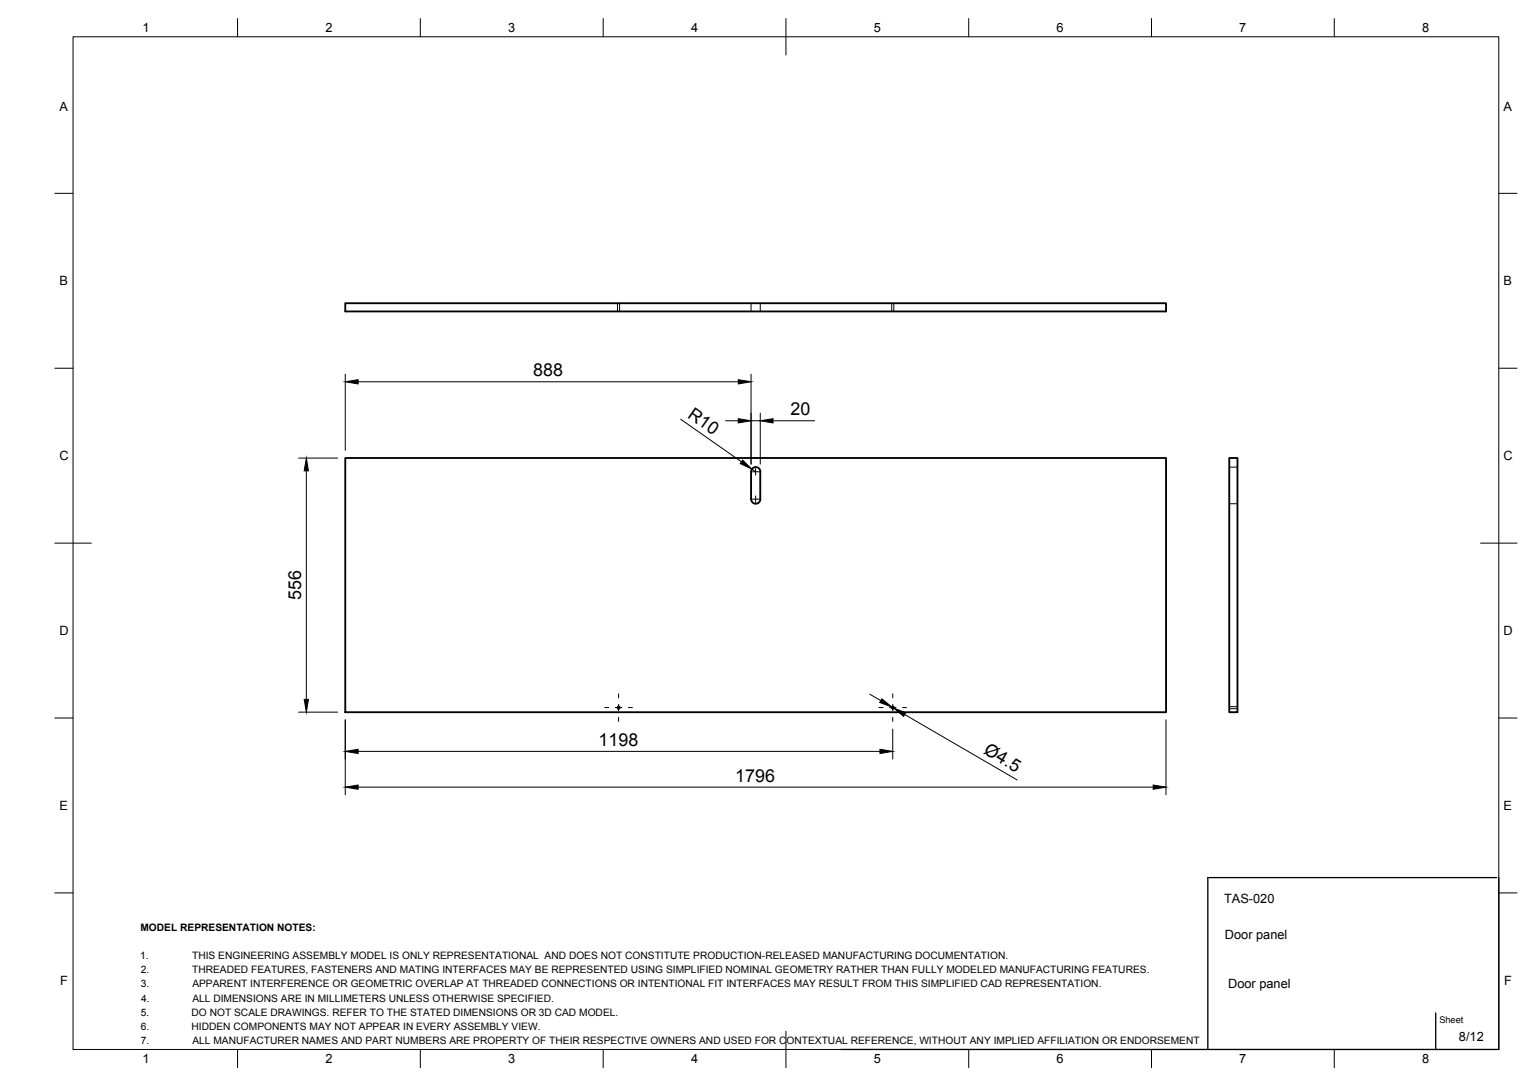
ISO-10303-21;
HEADER;
/* Generated by software containing ST-Developer
 * from STEP Tools, Inc. (www.steptools.com) 
 */

FILE_DESCRIPTION(
/* description */ (''),
/* implementation_level */ '2;1');

FILE_NAME(
/* name */ 'Door panel.step',
/* time_stamp */ '2026-11-15T17:46:57-08:00',
/* author */ (''),
/* organization */ (''),
/* preprocessor_version */ 'ST-DEVELOPER v20.2',
/* originating_system */ 'Autodesk Translation Framework v15.17.0.0',
/* authorisation */ '');

FILE_SCHEMA (('AUTOMOTIVE_DESIGN { 1 0 10303 214 3 1 1 }'));
ENDSEC;

DATA;
#10=MECHANICAL_DESIGN_GEOMETRIC_PRESENTATION_REPRESENTATION('',(#380),#12963);
#356=SHAPE_REPRESENTATION_RELATIONSHIP('SRR','None',#13040,#368);
#368=ADVANCED_BREP_SHAPE_REPRESENTATION('',(#392),#12956);
#380=STYLED_ITEM('',(#13109),#392);
#392=MANIFOLD_SOLID_BREP('Body1',#4814);
#417=FACE_BOUND('',#945,.T.);
#418=FACE_BOUND('',#946,.T.);
#419=FACE_BOUND('',#947,.T.);
#420=FACE_BOUND('',#950,.T.);
#421=FACE_BOUND('',#951,.T.);
#422=FACE_BOUND('',#952,.T.);
#519=PLANE('',#5081);
#520=PLANE('',#5085);
#521=PLANE('',#5095);
#522=PLANE('',#5096);
#523=PLANE('',#5097);
#524=PLANE('',#5098);
#525=PLANE('',#5099);
#526=PLANE('',#5100);
#664=FACE_OUTER_BOUND('',#938,.T.);
#665=FACE_OUTER_BOUND('',#939,.T.);
#666=FACE_OUTER_BOUND('',#940,.T.);
#667=FACE_OUTER_BOUND('',#941,.T.);
#668=FACE_OUTER_BOUND('',#942,.T.);
#669=FACE_OUTER_BOUND('',#943,.T.);
#670=FACE_OUTER_BOUND('',#944,.T.);
#671=FACE_OUTER_BOUND('',#948,.T.);
#672=FACE_OUTER_BOUND('',#949,.T.);
#673=FACE_OUTER_BOUND('',#953,.T.);
#674=FACE_OUTER_BOUND('',#954,.T.);
#675=FACE_OUTER_BOUND('',#955,.T.);
#938=EDGE_LOOP('',(#3544,#3545,#3546,#3547));
#939=EDGE_LOOP('',(#3548,#3549,#3550,#3551));
#940=EDGE_LOOP('',(#3552,#3553,#3554,#3555));
#941=EDGE_LOOP('',(#3556,#3557,#3558,#3559));
#942=EDGE_LOOP('',(#3560,#3561,#3562,#3563));
#943=EDGE_LOOP('',(#3564,#3565,#3566,#3567));
#944=EDGE_LOOP('',(#3568,#3569,#3570,#3571));
#945=EDGE_LOOP('',(#3572,#3573,#3574,#3575));
#946=EDGE_LOOP('',(#3576));
#947=EDGE_LOOP('',(#3577));
#948=EDGE_LOOP('',(#3578,#3579,#3580,#3581));
#949=EDGE_LOOP('',(#3582,#3583,#3584,#3585));
#950=EDGE_LOOP('',(#3586,#3587,#3588,#3589));
#951=EDGE_LOOP('',(#3590));
#952=EDGE_LOOP('',(#3591));
#953=EDGE_LOOP('',(#3592,#3593,#3594,#3595));
#954=EDGE_LOOP('',(#3596,#3597,#3598,#3599));
#955=EDGE_LOOP('',(#3600,#3601,#3602,#3603));
#1314=LINE('',#6979,#1716);
#1315=LINE('',#6981,#1717);
#1316=LINE('',#6983,#1718);
#1317=LINE('',#6984,#1719);
#1318=LINE('',#6989,#1720);
#1319=LINE('',#6993,#1721);
#1320=LINE('',#6995,#1722);
#1321=LINE('',#6996,#1723);
#1322=LINE('',#7004,#1724);
#1323=LINE('',#7010,#1725);
#1324=LINE('',#7015,#1726);
#1325=LINE('',#7017,#1727);
#1326=LINE('',#7019,#1728);
#1327=LINE('',#7020,#1729);
#1328=LINE('',#7023,#1730);
#1329=LINE('',#7025,#1731);
#1330=LINE('',#7026,#1732);
#1331=LINE('',#7029,#1733);
#1332=LINE('',#7031,#1734);
#1333=LINE('',#7032,#1735);
#1334=LINE('',#7034,#1736);
#1335=LINE('',#7035,#1737);
#1716=VECTOR('',#5785,1.);
#1717=VECTOR('',#5786,1.);
#1718=VECTOR('',#5787,1.);
#1719=VECTOR('',#5788,1.);
#1720=VECTOR('',#5793,1.);
#1721=VECTOR('',#5798,1.);
#1722=VECTOR('',#5799,1.);
#1723=VECTOR('',#5800,1.);
#1724=VECTOR('',#5811,0.225);
#1725=VECTOR('',#5818,0.225);
#1726=VECTOR('',#5823,1.);
#1727=VECTOR('',#5824,1.);
#1728=VECTOR('',#5825,1.);
#1729=VECTOR('',#5826,1.);
#1730=VECTOR('',#5829,1.);
#1731=VECTOR('',#5830,1.);
#1732=VECTOR('',#5831,1.);
#1733=VECTOR('',#5834,1.);
#1734=VECTOR('',#5835,1.);
#1735=VECTOR('',#5836,1.);
#1736=VECTOR('',#5839,1.);
#1737=VECTOR('',#5840,1.);
#1958=CIRCLE('',#5083,1.);
#1959=CIRCLE('',#5084,1.);
#1960=CIRCLE('',#5087,1.);
#1961=CIRCLE('',#5088,1.);
#1962=CIRCLE('',#5090,0.225);
#1963=CIRCLE('',#5091,0.225);
#1964=CIRCLE('',#5093,0.225);
#1965=CIRCLE('',#5094,0.225);
#2156=VERTEX_POINT('',#6977);
#2157=VERTEX_POINT('',#6978);
#2158=VERTEX_POINT('',#6980);
#2159=VERTEX_POINT('',#6982);
#2160=VERTEX_POINT('',#6986);
#2161=VERTEX_POINT('',#6988);
#2162=VERTEX_POINT('',#6992);
#2163=VERTEX_POINT('',#6994);
#2164=VERTEX_POINT('',#7001);
#2165=VERTEX_POINT('',#7003);
#2166=VERTEX_POINT('',#7007);
#2167=VERTEX_POINT('',#7009);
#2168=VERTEX_POINT('',#7013);
#2169=VERTEX_POINT('',#7014);
#2170=VERTEX_POINT('',#7016);
#2171=VERTEX_POINT('',#7018);
#2172=VERTEX_POINT('',#7022);
#2173=VERTEX_POINT('',#7024);
#2174=VERTEX_POINT('',#7028);
#2175=VERTEX_POINT('',#7030);
#2668=EDGE_CURVE('',#2156,#2157,#1314,.T.);
#2669=EDGE_CURVE('',#2156,#2158,#1315,.T.);
#2670=EDGE_CURVE('',#2159,#2158,#1316,.T.);
#2671=EDGE_CURVE('',#2157,#2159,#1317,.T.);
#2672=EDGE_CURVE('',#2160,#2156,#1958,.T.);
#2673=EDGE_CURVE('',#2160,#2161,#1318,.T.);
#2674=EDGE_CURVE('',#2158,#2161,#1959,.T.);
#2675=EDGE_CURVE('',#2162,#2160,#1319,.T.);
#2676=EDGE_CURVE('',#2162,#2163,#1320,.T.);
#2677=EDGE_CURVE('',#2161,#2163,#1321,.T.);
#2678=EDGE_CURVE('',#2157,#2162,#1960,.T.);
#2679=EDGE_CURVE('',#2163,#2159,#1961,.T.);
#2680=EDGE_CURVE('',#2164,#2164,#1962,.T.);
#2681=EDGE_CURVE('',#2164,#2165,#1322,.T.);
#2682=EDGE_CURVE('',#2165,#2165,#1963,.T.);
#2683=EDGE_CURVE('',#2166,#2166,#1964,.T.);
#2684=EDGE_CURVE('',#2166,#2167,#1323,.T.);
#2685=EDGE_CURVE('',#2167,#2167,#1965,.T.);
#2686=EDGE_CURVE('',#2168,#2169,#1324,.T.);
#2687=EDGE_CURVE('',#2169,#2170,#1325,.T.);
#2688=EDGE_CURVE('',#2171,#2170,#1326,.T.);
#2689=EDGE_CURVE('',#2168,#2171,#1327,.T.);
#2690=EDGE_CURVE('',#2172,#2168,#1328,.T.);
#2691=EDGE_CURVE('',#2173,#2171,#1329,.T.);
#2692=EDGE_CURVE('',#2172,#2173,#1330,.T.);
#2693=EDGE_CURVE('',#2174,#2172,#1331,.T.);
#2694=EDGE_CURVE('',#2175,#2173,#1332,.T.);
#2695=EDGE_CURVE('',#2174,#2175,#1333,.T.);
#2696=EDGE_CURVE('',#2169,#2174,#1334,.T.);
#2697=EDGE_CURVE('',#2170,#2175,#1335,.T.);
#3544=ORIENTED_EDGE('',*,*,#2668,.F.);
#3545=ORIENTED_EDGE('',*,*,#2669,.T.);
#3546=ORIENTED_EDGE('',*,*,#2670,.F.);
#3547=ORIENTED_EDGE('',*,*,#2671,.F.);
#3548=ORIENTED_EDGE('',*,*,#2672,.F.);
#3549=ORIENTED_EDGE('',*,*,#2673,.T.);
#3550=ORIENTED_EDGE('',*,*,#2674,.F.);
#3551=ORIENTED_EDGE('',*,*,#2669,.F.);
#3552=ORIENTED_EDGE('',*,*,#2675,.F.);
#3553=ORIENTED_EDGE('',*,*,#2676,.T.);
#3554=ORIENTED_EDGE('',*,*,#2677,.F.);
#3555=ORIENTED_EDGE('',*,*,#2673,.F.);
#3556=ORIENTED_EDGE('',*,*,#2678,.F.);
#3557=ORIENTED_EDGE('',*,*,#2671,.T.);
#3558=ORIENTED_EDGE('',*,*,#2679,.F.);
#3559=ORIENTED_EDGE('',*,*,#2676,.F.);
#3560=ORIENTED_EDGE('',*,*,#2680,.F.);
#3561=ORIENTED_EDGE('',*,*,#2681,.T.);
#3562=ORIENTED_EDGE('',*,*,#2682,.F.);
#3563=ORIENTED_EDGE('',*,*,#2681,.F.);
#3564=ORIENTED_EDGE('',*,*,#2683,.F.);
#3565=ORIENTED_EDGE('',*,*,#2684,.T.);
#3566=ORIENTED_EDGE('',*,*,#2685,.F.);
#3567=ORIENTED_EDGE('',*,*,#2684,.F.);
#3568=ORIENTED_EDGE('',*,*,#2686,.T.);
#3569=ORIENTED_EDGE('',*,*,#2687,.T.);
#3570=ORIENTED_EDGE('',*,*,#2688,.F.);
#3571=ORIENTED_EDGE('',*,*,#2689,.F.);
#3572=ORIENTED_EDGE('',*,*,#2668,.T.);
#3573=ORIENTED_EDGE('',*,*,#2678,.T.);
#3574=ORIENTED_EDGE('',*,*,#2675,.T.);
#3575=ORIENTED_EDGE('',*,*,#2672,.T.);
#3576=ORIENTED_EDGE('',*,*,#2680,.T.);
#3577=ORIENTED_EDGE('',*,*,#2683,.T.);
#3578=ORIENTED_EDGE('',*,*,#2690,.T.);
#3579=ORIENTED_EDGE('',*,*,#2689,.T.);
#3580=ORIENTED_EDGE('',*,*,#2691,.F.);
#3581=ORIENTED_EDGE('',*,*,#2692,.F.);
#3582=ORIENTED_EDGE('',*,*,#2693,.T.);
#3583=ORIENTED_EDGE('',*,*,#2692,.T.);
#3584=ORIENTED_EDGE('',*,*,#2694,.F.);
#3585=ORIENTED_EDGE('',*,*,#2695,.F.);
#3586=ORIENTED_EDGE('',*,*,#2670,.T.);
#3587=ORIENTED_EDGE('',*,*,#2674,.T.);
#3588=ORIENTED_EDGE('',*,*,#2677,.T.);
#3589=ORIENTED_EDGE('',*,*,#2679,.T.);
#3590=ORIENTED_EDGE('',*,*,#2682,.T.);
#3591=ORIENTED_EDGE('',*,*,#2685,.T.);
#3592=ORIENTED_EDGE('',*,*,#2696,.T.);
#3593=ORIENTED_EDGE('',*,*,#2695,.T.);
#3594=ORIENTED_EDGE('',*,*,#2697,.F.);
#3595=ORIENTED_EDGE('',*,*,#2687,.F.);
#3596=ORIENTED_EDGE('',*,*,#2697,.T.);
#3597=ORIENTED_EDGE('',*,*,#2694,.T.);
#3598=ORIENTED_EDGE('',*,*,#2691,.T.);
#3599=ORIENTED_EDGE('',*,*,#2688,.T.);
#3600=ORIENTED_EDGE('',*,*,#2696,.F.);
#3601=ORIENTED_EDGE('',*,*,#2686,.F.);
#3602=ORIENTED_EDGE('',*,*,#2690,.F.);
#3603=ORIENTED_EDGE('',*,*,#2693,.F.);
#4446=CYLINDRICAL_SURFACE('',#5082,1.);
#4447=CYLINDRICAL_SURFACE('',#5086,1.);
#4448=CYLINDRICAL_SURFACE('',#5089,0.225);
#4449=CYLINDRICAL_SURFACE('',#5092,0.225);
#4645=ADVANCED_FACE('',(#664),#519,.F.);
#4646=ADVANCED_FACE('',(#665),#4446,.F.);
#4647=ADVANCED_FACE('',(#666),#520,.F.);
#4648=ADVANCED_FACE('',(#667),#4447,.F.);
#4649=ADVANCED_FACE('',(#668),#4448,.F.);
#4650=ADVANCED_FACE('',(#669),#4449,.F.);
#4651=ADVANCED_FACE('',(#670,#417,#418,#419),#521,.T.);
#4652=ADVANCED_FACE('',(#671),#522,.T.);
#4653=ADVANCED_FACE('',(#672,#420,#421,#422),#523,.T.);
#4654=ADVANCED_FACE('',(#673),#524,.T.);
#4655=ADVANCED_FACE('',(#674),#525,.T.);
#4656=ADVANCED_FACE('',(#675),#526,.F.);
#4814=CLOSED_SHELL('',(#4645,#4646,#4647,#4648,#4649,#4650,#4651,#4652,
#4653,#4654,#4655,#4656));
#5080=AXIS2_PLACEMENT_3D('',#6975,#5781,#5782);
#5081=AXIS2_PLACEMENT_3D('',#6976,#5783,#5784);
#5082=AXIS2_PLACEMENT_3D('',#6985,#5789,#5790);
#5083=AXIS2_PLACEMENT_3D('',#6987,#5791,#5792);
#5084=AXIS2_PLACEMENT_3D('',#6990,#5794,#5795);
#5085=AXIS2_PLACEMENT_3D('',#6991,#5796,#5797);
#5086=AXIS2_PLACEMENT_3D('',#6997,#5801,#5802);
#5087=AXIS2_PLACEMENT_3D('',#6998,#5803,#5804);
#5088=AXIS2_PLACEMENT_3D('',#6999,#5805,#5806);
#5089=AXIS2_PLACEMENT_3D('',#7000,#5807,#5808);
#5090=AXIS2_PLACEMENT_3D('',#7002,#5809,#5810);
#5091=AXIS2_PLACEMENT_3D('',#7005,#5812,#5813);
#5092=AXIS2_PLACEMENT_3D('',#7006,#5814,#5815);
#5093=AXIS2_PLACEMENT_3D('',#7008,#5816,#5817);
#5094=AXIS2_PLACEMENT_3D('',#7011,#5819,#5820);
#5095=AXIS2_PLACEMENT_3D('',#7012,#5821,#5822);
#5096=AXIS2_PLACEMENT_3D('',#7021,#5827,#5828);
#5097=AXIS2_PLACEMENT_3D('',#7027,#5832,#5833);
#5098=AXIS2_PLACEMENT_3D('',#7033,#5837,#5838);
#5099=AXIS2_PLACEMENT_3D('',#7036,#5841,#5842);
#5100=AXIS2_PLACEMENT_3D('',#7037,#5843,#5844);
#5781=DIRECTION('axis',(0.,0.,1.));
#5782=DIRECTION('refdir',(1.,0.,0.));
#5783=DIRECTION('center_axis',(0.,0.,-1.));
#5784=DIRECTION('ref_axis',(1.,0.,0.));
#5785=DIRECTION('',(1.,0.,0.));
#5786=DIRECTION('',(0.,-1.,0.));
#5787=DIRECTION('',(-1.,0.,0.));
#5788=DIRECTION('',(0.,-1.,0.));
#5789=DIRECTION('center_axis',(0.,-1.,0.));
#5790=DIRECTION('ref_axis',(0.,0.,-1.));
#5791=DIRECTION('center_axis',(0.,-1.,0.));
#5792=DIRECTION('ref_axis',(0.,0.,-1.));
#5793=DIRECTION('',(0.,-1.,0.));
#5794=DIRECTION('center_axis',(0.,1.,0.));
#5795=DIRECTION('ref_axis',(0.,0.,-1.));
#5796=DIRECTION('center_axis',(0.,0.,1.));
#5797=DIRECTION('ref_axis',(-1.,0.,0.));
#5798=DIRECTION('',(-1.,0.,0.));
#5799=DIRECTION('',(0.,-1.,0.));
#5800=DIRECTION('',(1.,0.,0.));
#5801=DIRECTION('center_axis',(0.,-1.,0.));
#5802=DIRECTION('ref_axis',(0.,0.,1.));
#5803=DIRECTION('center_axis',(0.,-1.,0.));
#5804=DIRECTION('ref_axis',(0.,0.,1.));
#5805=DIRECTION('center_axis',(0.,1.,0.));
#5806=DIRECTION('ref_axis',(0.,0.,1.));
#5807=DIRECTION('center_axis',(0.,-1.,0.));
#5808=DIRECTION('ref_axis',(1.,0.,0.));
#5809=DIRECTION('center_axis',(0.,-1.,0.));
#5810=DIRECTION('ref_axis',(1.,0.,0.));
#5811=DIRECTION('',(0.,-1.,0.));
#5812=DIRECTION('center_axis',(0.,1.,0.));
#5813=DIRECTION('ref_axis',(1.,0.,0.));
#5814=DIRECTION('center_axis',(0.,-1.,0.));
#5815=DIRECTION('ref_axis',(1.,0.,0.));
#5816=DIRECTION('center_axis',(0.,-1.,0.));
#5817=DIRECTION('ref_axis',(1.,0.,0.));
#5818=DIRECTION('',(0.,-1.,0.));
#5819=DIRECTION('center_axis',(0.,1.,0.));
#5820=DIRECTION('ref_axis',(1.,0.,0.));
#5821=DIRECTION('center_axis',(0.,1.,0.));
#5822=DIRECTION('ref_axis',(-1.,0.,0.));
#5823=DIRECTION('',(-1.,0.,0.));
#5824=DIRECTION('',(0.,0.,1.));
#5825=DIRECTION('',(-1.,0.,0.));
#5826=DIRECTION('',(0.,0.,1.));
#5827=DIRECTION('center_axis',(1.,0.,0.));
#5828=DIRECTION('ref_axis',(0.,1.,0.));
#5829=DIRECTION('',(0.,1.,0.));
#5830=DIRECTION('',(0.,1.,0.));
#5831=DIRECTION('',(0.,0.,1.));
#5832=DIRECTION('center_axis',(0.,-1.,0.));
#5833=DIRECTION('ref_axis',(1.,0.,0.));
#5834=DIRECTION('',(1.,0.,0.));
#5835=DIRECTION('',(1.,0.,0.));
#5836=DIRECTION('',(0.,0.,1.));
#5837=DIRECTION('center_axis',(-1.,0.,0.));
#5838=DIRECTION('ref_axis',(0.,-1.,0.));
#5839=DIRECTION('',(0.,-1.,0.));
#5840=DIRECTION('',(0.,-1.,0.));
#5841=DIRECTION('center_axis',(0.,0.,1.));
#5842=DIRECTION('ref_axis',(1.,0.,0.));
#5843=DIRECTION('center_axis',(0.,0.,1.));
#5844=DIRECTION('ref_axis',(1.,0.,0.));
#6975=CARTESIAN_POINT('',(0.,0.,0.));
#6976=CARTESIAN_POINT('Origin',(49.,-0.2,89.));
#6977=CARTESIAN_POINT('',(49.,-0.2,89.));
#6978=CARTESIAN_POINT('',(55.,-0.2,89.));
#6979=CARTESIAN_POINT('',(53.5,-0.2,89.));
#6980=CARTESIAN_POINT('',(49.,-2.,89.));
#6981=CARTESIAN_POINT('',(49.,-0.2,89.));
#6982=CARTESIAN_POINT('',(55.,-2.,89.));
#6983=CARTESIAN_POINT('',(25.7,-2.,89.));
#6984=CARTESIAN_POINT('',(55.,-0.2,89.));
#6985=CARTESIAN_POINT('Origin',(49.,-0.2,90.));
#6986=CARTESIAN_POINT('',(49.,-0.2,91.));
#6987=CARTESIAN_POINT('Origin',(49.,-0.2,90.));
#6988=CARTESIAN_POINT('',(49.,-2.,91.));
#6989=CARTESIAN_POINT('',(49.,-0.2,91.));
#6990=CARTESIAN_POINT('Origin',(49.,-2.,90.));
#6991=CARTESIAN_POINT('Origin',(55.,-0.2,91.));
#6992=CARTESIAN_POINT('',(55.,-0.2,91.));
#6993=CARTESIAN_POINT('',(56.5,-0.2,91.));
#6994=CARTESIAN_POINT('',(55.,-2.,91.));
#6995=CARTESIAN_POINT('',(55.,-0.2,91.));
#6996=CARTESIAN_POINT('',(28.7,-2.,91.));
#6997=CARTESIAN_POINT('Origin',(55.,-0.2,90.));
#6998=CARTESIAN_POINT('Origin',(55.,-0.2,90.));
#6999=CARTESIAN_POINT('Origin',(55.,-2.,90.));
#7000=CARTESIAN_POINT('Origin',(3.4,-0.2,60.));
#7001=CARTESIAN_POINT('',(3.175,-0.2,60.));
#7002=CARTESIAN_POINT('Origin',(3.4,-0.2,60.));
#7003=CARTESIAN_POINT('',(3.175,-2.,60.));
#7004=CARTESIAN_POINT('',(3.175,-0.2,60.));
#7005=CARTESIAN_POINT('Origin',(3.4,-2.,60.));
#7006=CARTESIAN_POINT('Origin',(3.4,-0.2,120.));
#7007=CARTESIAN_POINT('',(3.175,-0.2,120.));
#7008=CARTESIAN_POINT('Origin',(3.4,-0.2,120.));
#7009=CARTESIAN_POINT('',(3.175,-2.,120.));
#7010=CARTESIAN_POINT('',(3.175,-0.2,120.));
#7011=CARTESIAN_POINT('Origin',(3.4,-2.,120.));
#7012=CARTESIAN_POINT('Origin',(58.,-0.2,0.2));
#7013=CARTESIAN_POINT('',(58.,-0.2,0.2));
#7014=CARTESIAN_POINT('',(2.4,-0.2,0.2));
#7015=CARTESIAN_POINT('',(58.,-0.2,0.2));
#7016=CARTESIAN_POINT('',(2.4,-0.2,179.8));
#7017=CARTESIAN_POINT('',(2.4,-0.2,0.2));
#7018=CARTESIAN_POINT('',(58.,-0.2,179.8));
#7019=CARTESIAN_POINT('',(58.,-0.2,179.8));
#7020=CARTESIAN_POINT('',(58.,-0.2,0.2));
#7021=CARTESIAN_POINT('Origin',(58.,-2.,0.2));
#7022=CARTESIAN_POINT('',(58.,-2.,0.2));
#7023=CARTESIAN_POINT('',(58.,-2.,0.2));
#7024=CARTESIAN_POINT('',(58.,-2.,179.8));
#7025=CARTESIAN_POINT('',(58.,-2.,179.8));
#7026=CARTESIAN_POINT('',(58.,-2.,0.2));
#7027=CARTESIAN_POINT('Origin',(2.4,-2.,0.2));
#7028=CARTESIAN_POINT('',(2.4,-2.,0.2));
#7029=CARTESIAN_POINT('',(2.4,-2.,0.2));
#7030=CARTESIAN_POINT('',(2.4,-2.,179.8));
#7031=CARTESIAN_POINT('',(2.4,-2.,179.8));
#7032=CARTESIAN_POINT('',(2.4,-2.,0.2));
#7033=CARTESIAN_POINT('Origin',(2.4,-0.2,0.2));
#7034=CARTESIAN_POINT('',(2.4,-0.2,0.2));
#7035=CARTESIAN_POINT('',(2.4,-0.2,179.8));
#7036=CARTESIAN_POINT('Origin',(30.2,-1.1,179.8));
#7037=CARTESIAN_POINT('Origin',(30.2,-1.1,0.2));
#12942=UNCERTAINTY_MEASURE_WITH_UNIT(LENGTH_MEASURE(0.001),#12964,
'DISTANCE_ACCURACY_VALUE',
'Maximum model space distance between geometric entities at asserted c
onnectivities');
#12949=UNCERTAINTY_MEASURE_WITH_UNIT(LENGTH_MEASURE(0.001),#12964,
'DISTANCE_ACCURACY_VALUE',
'Maximum model space distance between geometric entities at asserted c
onnectivities');
#12956=(
GEOMETRIC_REPRESENTATION_CONTEXT(3)
GLOBAL_UNCERTAINTY_ASSIGNED_CONTEXT((#12942))
GLOBAL_UNIT_ASSIGNED_CONTEXT((#12964,#12966,#12967))
REPRESENTATION_CONTEXT('','3D')
);
#12963=(
GEOMETRIC_REPRESENTATION_CONTEXT(3)
GLOBAL_UNCERTAINTY_ASSIGNED_CONTEXT((#12949))
GLOBAL_UNIT_ASSIGNED_CONTEXT((#12964,#12966,#12967))
REPRESENTATION_CONTEXT('','3D')
);
#12964=(
LENGTH_UNIT()
NAMED_UNIT(*)
SI_UNIT(.CENTI.,.METRE.)
);
#12966=(
NAMED_UNIT(*)
PLANE_ANGLE_UNIT()
SI_UNIT($,.RADIAN.)
);
#12967=(
NAMED_UNIT(*)
SI_UNIT($,.STERADIAN.)
SOLID_ANGLE_UNIT()
);
#12974=SHAPE_DEFINITION_REPRESENTATION(#12987,#13040);
#12987=PRODUCT_DEFINITION_SHAPE('',$,#13054);
#13040=SHAPE_REPRESENTATION('',(#5080),#12956);
#13047=PRODUCT_DEFINITION_CONTEXT('part definition',#13088,'design');
#13054=PRODUCT_DEFINITION('Door panel','Door panel',#13067,#13047);
#13067=PRODUCT_DEFINITION_FORMATION('',$,#13096);
#13088=APPLICATION_CONTEXT(
'Core Data for Automotive Mechanical Design Process');
#13089=PRODUCT_CONTEXT('part definition',#13088,'mechanical');
#13096=PRODUCT('Door panel','Door panel','Door panel',(#13089));
#13109=PRESENTATION_STYLE_ASSIGNMENT((#13122));
#13122=SURFACE_STYLE_USAGE(.BOTH.,#13135);
#13135=SURFACE_SIDE_STYLE('',(#13148));
#13148=SURFACE_STYLE_FILL_AREA(#13161);
#13161=FILL_AREA_STYLE('Door panel finish',(#13174));
#13174=FILL_AREA_STYLE_COLOUR('Door panel finish',#13187);
#13187=COLOUR_RGB('Door panel finish',0.274509803921569,0.6,0.8);
ENDSEC;
END-ISO-10303-21;
